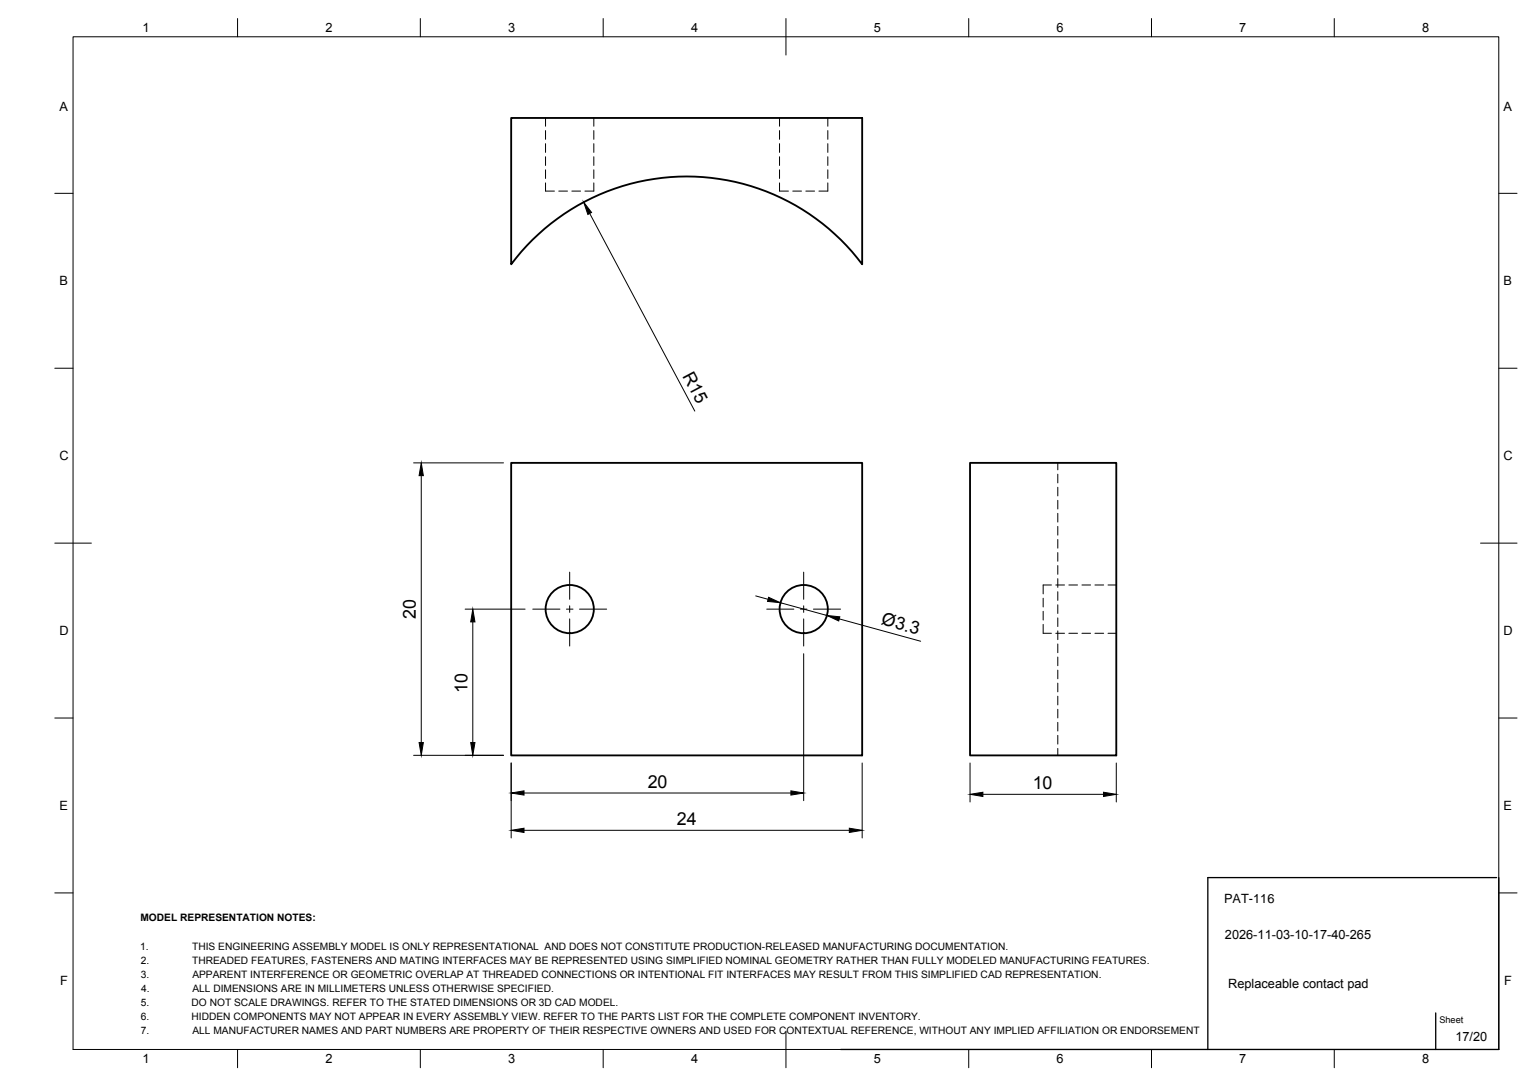
ISO-10303-21;
HEADER;
/* Generated by software containing ST-Developer
 * from STEP Tools, Inc. (www.steptools.com) 
 */

FILE_DESCRIPTION(
/* description */ ('V-block with clamp strap'),
/* implementation_level */ '2;1');

FILE_NAME(
/* name */ 'Replaceable contact pad.step',
/* time_stamp */ '2026-10-27T10:50:53-07:00',
/* author */ (''),
/* organization */ (''),
/* preprocessor_version */ 'ST-DEVELOPER v20.2',
/* originating_system */ 'Autodesk Translation Framework v15.17.0.0',
/* authorisation */ '');

FILE_SCHEMA (('AUTOMOTIVE_DESIGN { 1 0 10303 214 3 1 1 }'));
ENDSEC;

DATA;
#10=MECHANICAL_DESIGN_GEOMETRIC_PRESENTATION_REPRESENTATION('',(#280),#7344);
#238=SHAPE_REPRESENTATION_RELATIONSHIP('SRR','None',#7457,#259);
#259=ADVANCED_BREP_SHAPE_REPRESENTATION('',(#299),#7336);
#280=STYLED_ITEM('',(#7624),#299);
#299=MANIFOLD_SOLID_BREP('Body1',#4164);
#369=FACE_BOUND('',#1066,.T.);
#370=FACE_BOUND('',#1067,.T.);
#478=CIRCLE('',#4742,0.164999999999999);
#479=CIRCLE('',#4743,0.164999999999999);
#480=CIRCLE('',#4746,0.164999999999999);
#481=CIRCLE('',#4747,0.164999999999999);
#482=CIRCLE('',#4750,1.5);
#483=CIRCLE('',#4751,1.5);
#551=CYLINDRICAL_SURFACE('',#4741,0.164999999999999);
#552=CYLINDRICAL_SURFACE('',#4745,0.164999999999999);
#553=CYLINDRICAL_SURFACE('',#4749,1.5);
#752=FACE_OUTER_BOUND('',#1056,.T.);
#753=FACE_OUTER_BOUND('',#1057,.T.);
#754=FACE_OUTER_BOUND('',#1058,.T.);
#755=FACE_OUTER_BOUND('',#1059,.T.);
#756=FACE_OUTER_BOUND('',#1060,.T.);
#757=FACE_OUTER_BOUND('',#1061,.T.);
#758=FACE_OUTER_BOUND('',#1062,.T.);
#759=FACE_OUTER_BOUND('',#1063,.T.);
#760=FACE_OUTER_BOUND('',#1064,.T.);
#761=FACE_OUTER_BOUND('',#1065,.T.);
#1056=EDGE_LOOP('',(#3564,#3565,#3566,#3567));
#1057=EDGE_LOOP('',(#3568));
#1058=EDGE_LOOP('',(#3569,#3570,#3571,#3572));
#1059=EDGE_LOOP('',(#3573));
#1060=EDGE_LOOP('',(#3574,#3575,#3576,#3577));
#1061=EDGE_LOOP('',(#3578,#3579,#3580,#3581));
#1062=EDGE_LOOP('',(#3582,#3583,#3584,#3585));
#1063=EDGE_LOOP('',(#3586,#3587,#3588,#3589));
#1064=EDGE_LOOP('',(#3590,#3591,#3592,#3593));
#1065=EDGE_LOOP('',(#3594,#3595,#3596,#3597));
#1066=EDGE_LOOP('',(#3598));
#1067=EDGE_LOOP('',(#3599));
#1429=LINE('',#7053,#1794);
#1430=LINE('',#7060,#1795);
#1431=LINE('',#7066,#1796);
#1432=LINE('',#7070,#1797);
#1433=LINE('',#7074,#1798);
#1434=LINE('',#7076,#1799);
#1435=LINE('',#7077,#1800);
#1436=LINE('',#7080,#1801);
#1437=LINE('',#7081,#1802);
#1438=LINE('',#7084,#1803);
#1439=LINE('',#7085,#1804);
#1440=LINE('',#7087,#1805);
#1794=VECTOR('',#5837,0.164999999999999);
#1795=VECTOR('',#5846,0.164999999999999);
#1796=VECTOR('',#5853,1.);
#1797=VECTOR('',#5856,1.);
#1798=VECTOR('',#5861,1.);
#1799=VECTOR('',#5862,1.);
#1800=VECTOR('',#5863,1.);
#1801=VECTOR('',#5866,1.);
#1802=VECTOR('',#5867,1.);
#1803=VECTOR('',#5870,1.);
#1804=VECTOR('',#5871,1.);
#1805=VECTOR('',#5874,1.);
#2117=VERTEX_POINT('',#7050);
#2118=VERTEX_POINT('',#7052);
#2119=VERTEX_POINT('',#7057);
#2120=VERTEX_POINT('',#7059);
#2121=VERTEX_POINT('',#7064);
#2122=VERTEX_POINT('',#7065);
#2123=VERTEX_POINT('',#7067);
#2124=VERTEX_POINT('',#7069);
#2125=VERTEX_POINT('',#7073);
#2126=VERTEX_POINT('',#7075);
#2127=VERTEX_POINT('',#7079);
#2128=VERTEX_POINT('',#7083);
#2608=EDGE_CURVE('',#2117,#2117,#478,.T.);
#2609=EDGE_CURVE('',#2117,#2118,#1429,.T.);
#2610=EDGE_CURVE('',#2118,#2118,#479,.T.);
#2611=EDGE_CURVE('',#2119,#2119,#480,.T.);
#2612=EDGE_CURVE('',#2119,#2120,#1430,.T.);
#2613=EDGE_CURVE('',#2120,#2120,#481,.T.);
#2614=EDGE_CURVE('',#2121,#2122,#1431,.T.);
#2615=EDGE_CURVE('',#2123,#2121,#482,.T.);
#2616=EDGE_CURVE('',#2124,#2123,#1432,.T.);
#2617=EDGE_CURVE('',#2122,#2124,#483,.T.);
#2618=EDGE_CURVE('',#2121,#2125,#1433,.T.);
#2619=EDGE_CURVE('',#2126,#2125,#1434,.T.);
#2620=EDGE_CURVE('',#2123,#2126,#1435,.T.);
#2621=EDGE_CURVE('',#2122,#2127,#1436,.T.);
#2622=EDGE_CURVE('',#2125,#2127,#1437,.T.);
#2623=EDGE_CURVE('',#2128,#2126,#1438,.T.);
#2624=EDGE_CURVE('',#2124,#2128,#1439,.T.);
#2625=EDGE_CURVE('',#2127,#2128,#1440,.T.);
#3564=ORIENTED_EDGE('',*,*,#2608,.F.);
#3565=ORIENTED_EDGE('',*,*,#2609,.T.);
#3566=ORIENTED_EDGE('',*,*,#2610,.F.);
#3567=ORIENTED_EDGE('',*,*,#2609,.F.);
#3568=ORIENTED_EDGE('',*,*,#2608,.T.);
#3569=ORIENTED_EDGE('',*,*,#2611,.F.);
#3570=ORIENTED_EDGE('',*,*,#2612,.T.);
#3571=ORIENTED_EDGE('',*,*,#2613,.F.);
#3572=ORIENTED_EDGE('',*,*,#2612,.F.);
#3573=ORIENTED_EDGE('',*,*,#2611,.T.);
#3574=ORIENTED_EDGE('',*,*,#2614,.F.);
#3575=ORIENTED_EDGE('',*,*,#2615,.F.);
#3576=ORIENTED_EDGE('',*,*,#2616,.F.);
#3577=ORIENTED_EDGE('',*,*,#2617,.F.);
#3578=ORIENTED_EDGE('',*,*,#2615,.T.);
#3579=ORIENTED_EDGE('',*,*,#2618,.T.);
#3580=ORIENTED_EDGE('',*,*,#2619,.F.);
#3581=ORIENTED_EDGE('',*,*,#2620,.F.);
#3582=ORIENTED_EDGE('',*,*,#2614,.T.);
#3583=ORIENTED_EDGE('',*,*,#2621,.T.);
#3584=ORIENTED_EDGE('',*,*,#2622,.F.);
#3585=ORIENTED_EDGE('',*,*,#2618,.F.);
#3586=ORIENTED_EDGE('',*,*,#2616,.T.);
#3587=ORIENTED_EDGE('',*,*,#2620,.T.);
#3588=ORIENTED_EDGE('',*,*,#2623,.F.);
#3589=ORIENTED_EDGE('',*,*,#2624,.F.);
#3590=ORIENTED_EDGE('',*,*,#2617,.T.);
#3591=ORIENTED_EDGE('',*,*,#2624,.T.);
#3592=ORIENTED_EDGE('',*,*,#2625,.F.);
#3593=ORIENTED_EDGE('',*,*,#2621,.F.);
#3594=ORIENTED_EDGE('',*,*,#2625,.T.);
#3595=ORIENTED_EDGE('',*,*,#2623,.T.);
#3596=ORIENTED_EDGE('',*,*,#2619,.T.);
#3597=ORIENTED_EDGE('',*,*,#2622,.T.);
#3598=ORIENTED_EDGE('',*,*,#2610,.T.);
#3599=ORIENTED_EDGE('',*,*,#2613,.T.);
#3874=PLANE('',#4744);
#3875=PLANE('',#4748);
#3876=PLANE('',#4752);
#3877=PLANE('',#4753);
#3878=PLANE('',#4754);
#3879=PLANE('',#4755);
#3880=PLANE('',#4756);
#4098=ADVANCED_FACE('',(#752),#551,.F.);
#4099=ADVANCED_FACE('',(#753),#3874,.T.);
#4100=ADVANCED_FACE('',(#754),#552,.F.);
#4101=ADVANCED_FACE('',(#755),#3875,.T.);
#4102=ADVANCED_FACE('',(#756),#553,.F.);
#4103=ADVANCED_FACE('',(#757),#3876,.T.);
#4104=ADVANCED_FACE('',(#758),#3877,.T.);
#4105=ADVANCED_FACE('',(#759),#3878,.T.);
#4106=ADVANCED_FACE('',(#760),#3879,.T.);
#4107=ADVANCED_FACE('',(#761,#369,#370),#3880,.T.);
#4164=CLOSED_SHELL('',(#4098,#4099,#4100,#4101,#4102,#4103,#4104,#4105,
#4106,#4107));
#4740=AXIS2_PLACEMENT_3D('',#7048,#5831,#5832);
#4741=AXIS2_PLACEMENT_3D('',#7049,#5833,#5834);
#4742=AXIS2_PLACEMENT_3D('',#7051,#5835,#5836);
#4743=AXIS2_PLACEMENT_3D('',#7054,#5838,#5839);
#4744=AXIS2_PLACEMENT_3D('',#7055,#5840,#5841);
#4745=AXIS2_PLACEMENT_3D('',#7056,#5842,#5843);
#4746=AXIS2_PLACEMENT_3D('',#7058,#5844,#5845);
#4747=AXIS2_PLACEMENT_3D('',#7061,#5847,#5848);
#4748=AXIS2_PLACEMENT_3D('',#7062,#5849,#5850);
#4749=AXIS2_PLACEMENT_3D('',#7063,#5851,#5852);
#4750=AXIS2_PLACEMENT_3D('',#7068,#5854,#5855);
#4751=AXIS2_PLACEMENT_3D('',#7071,#5857,#5858);
#4752=AXIS2_PLACEMENT_3D('',#7072,#5859,#5860);
#4753=AXIS2_PLACEMENT_3D('',#7078,#5864,#5865);
#4754=AXIS2_PLACEMENT_3D('',#7082,#5868,#5869);
#4755=AXIS2_PLACEMENT_3D('',#7086,#5872,#5873);
#4756=AXIS2_PLACEMENT_3D('',#7088,#5875,#5876);
#5831=DIRECTION('axis',(0.,0.,1.));
#5832=DIRECTION('refdir',(1.,0.,0.));
#5833=DIRECTION('center_axis',(0.,0.,1.));
#5834=DIRECTION('ref_axis',(1.,0.,0.));
#5835=DIRECTION('center_axis',(0.,0.,1.));
#5836=DIRECTION('ref_axis',(1.,0.,0.));
#5837=DIRECTION('',(0.,0.,1.));
#5838=DIRECTION('center_axis',(0.,0.,-1.));
#5839=DIRECTION('ref_axis',(1.,0.,0.));
#5840=DIRECTION('center_axis',(0.,0.,1.));
#5841=DIRECTION('ref_axis',(1.,0.,0.));
#5842=DIRECTION('center_axis',(0.,0.,1.));
#5843=DIRECTION('ref_axis',(1.,0.,0.));
#5844=DIRECTION('center_axis',(0.,0.,1.));
#5845=DIRECTION('ref_axis',(1.,0.,0.));
#5846=DIRECTION('',(0.,0.,1.));
#5847=DIRECTION('center_axis',(0.,0.,-1.));
#5848=DIRECTION('ref_axis',(1.,0.,0.));
#5849=DIRECTION('center_axis',(0.,0.,1.));
#5850=DIRECTION('ref_axis',(1.,0.,0.));
#5851=DIRECTION('center_axis',(1.,0.,0.));
#5852=DIRECTION('ref_axis',(0.,1.22464679914735E-16,1.));
#5853=DIRECTION('',(-1.,0.,0.));
#5854=DIRECTION('center_axis',(-1.,0.,0.));
#5855=DIRECTION('ref_axis',(0.,0.,-1.));
#5856=DIRECTION('',(1.,0.,0.));
#5857=DIRECTION('center_axis',(1.,0.,0.));
#5858=DIRECTION('ref_axis',(0.,0.,-1.));
#5859=DIRECTION('center_axis',(1.,0.,0.));
#5860=DIRECTION('ref_axis',(0.,1.,0.));
#5861=DIRECTION('',(0.,0.,1.));
#5862=DIRECTION('',(0.,1.,0.));
#5863=DIRECTION('',(0.,0.,1.));
#5864=DIRECTION('center_axis',(0.,1.,0.));
#5865=DIRECTION('ref_axis',(-1.,0.,0.));
#5866=DIRECTION('',(0.,0.,1.));
#5867=DIRECTION('',(-1.,0.,0.));
#5868=DIRECTION('center_axis',(0.,-1.,0.));
#5869=DIRECTION('ref_axis',(1.,0.,0.));
#5870=DIRECTION('',(1.,0.,0.));
#5871=DIRECTION('',(0.,0.,1.));
#5872=DIRECTION('center_axis',(-1.,0.,0.));
#5873=DIRECTION('ref_axis',(0.,-1.,0.));
#5874=DIRECTION('',(0.,-1.,0.));
#5875=DIRECTION('center_axis',(0.,0.,1.));
#5876=DIRECTION('ref_axis',(1.,0.,0.));
#7048=CARTESIAN_POINT('',(0.,0.,0.));
#7049=CARTESIAN_POINT('Origin',(10.,-0.8,6.02132034));
#7050=CARTESIAN_POINT('',(9.835,-0.8,6.02132034));
#7051=CARTESIAN_POINT('Origin',(10.,-0.8,6.02132034));
#7052=CARTESIAN_POINT('',(9.835,-0.8,6.52132034));
#7053=CARTESIAN_POINT('',(9.835,-0.8,6.02132034));
#7054=CARTESIAN_POINT('Origin',(10.,-0.8,6.52132034));
#7055=CARTESIAN_POINT('Origin',(10.,-0.8,6.02132034));
#7056=CARTESIAN_POINT('Origin',(10.,0.8,6.02132034));
#7057=CARTESIAN_POINT('',(9.835,0.8,6.02132034));
#7058=CARTESIAN_POINT('Origin',(10.,0.8,6.02132034));
#7059=CARTESIAN_POINT('',(9.835,0.8,6.52132034));
#7060=CARTESIAN_POINT('',(9.835,0.8,6.02132034));
#7061=CARTESIAN_POINT('Origin',(10.,0.8,6.52132034));
#7062=CARTESIAN_POINT('Origin',(10.,0.8,6.02132034));
#7063=CARTESIAN_POINT('Origin',(8.9,0.,4.62132034355964));
#7064=CARTESIAN_POINT('',(11.,1.2,5.52132034));
#7065=CARTESIAN_POINT('',(9.,1.2,5.52132034));
#7066=CARTESIAN_POINT('',(11.,1.2,5.52132034));
#7067=CARTESIAN_POINT('',(11.,-1.2,5.52132034));
#7068=CARTESIAN_POINT('Origin',(11.,0.,4.62132034355964));
#7069=CARTESIAN_POINT('',(9.,-1.2,5.52132034));
#7070=CARTESIAN_POINT('',(9.,-1.2,5.52132034));
#7071=CARTESIAN_POINT('Origin',(9.,0.,4.62132034355964));
#7072=CARTESIAN_POINT('Origin',(11.,-1.2,5.52132034));
#7073=CARTESIAN_POINT('',(11.,1.2,6.52132034));
#7074=CARTESIAN_POINT('',(11.,1.2,5.52132034));
#7075=CARTESIAN_POINT('',(11.,-1.2,6.52132034));
#7076=CARTESIAN_POINT('',(11.,-1.2,6.52132034));
#7077=CARTESIAN_POINT('',(11.,-1.2,5.52132034));
#7078=CARTESIAN_POINT('Origin',(11.,1.2,5.52132034));
#7079=CARTESIAN_POINT('',(9.,1.2,6.52132034));
#7080=CARTESIAN_POINT('',(9.,1.2,5.52132034));
#7081=CARTESIAN_POINT('',(11.,1.2,6.52132034));
#7082=CARTESIAN_POINT('Origin',(9.,-1.2,5.52132034));
#7083=CARTESIAN_POINT('',(9.,-1.2,6.52132034));
#7084=CARTESIAN_POINT('',(9.,-1.2,6.52132034));
#7085=CARTESIAN_POINT('',(9.,-1.2,5.52132034));
#7086=CARTESIAN_POINT('Origin',(9.,1.2,5.52132034));
#7087=CARTESIAN_POINT('',(9.,1.2,6.52132034));
#7088=CARTESIAN_POINT('Origin',(10.,0.,6.52132034));
#7310=UNCERTAINTY_MEASURE_WITH_UNIT(LENGTH_MEASURE(0.001),#7345,
'DISTANCE_ACCURACY_VALUE',
'Maximum model space distance between geometric entities at asserted c
onnectivities');
#7318=UNCERTAINTY_MEASURE_WITH_UNIT(LENGTH_MEASURE(0.001),#7345,
'DISTANCE_ACCURACY_VALUE',
'Maximum model space distance between geometric entities at asserted c
onnectivities');
#7336=(
GEOMETRIC_REPRESENTATION_CONTEXT(3)
GLOBAL_UNCERTAINTY_ASSIGNED_CONTEXT((#7310))
GLOBAL_UNIT_ASSIGNED_CONTEXT((#7345,#7347,#7348))
REPRESENTATION_CONTEXT('','3D')
);
#7344=(
GEOMETRIC_REPRESENTATION_CONTEXT(3)
GLOBAL_UNCERTAINTY_ASSIGNED_CONTEXT((#7318))
GLOBAL_UNIT_ASSIGNED_CONTEXT((#7345,#7347,#7348))
REPRESENTATION_CONTEXT('','3D')
);
#7345=(
LENGTH_UNIT()
NAMED_UNIT(*)
SI_UNIT(.CENTI.,.METRE.)
);
#7347=(
NAMED_UNIT(*)
PLANE_ANGLE_UNIT()
SI_UNIT($,.RADIAN.)
);
#7348=(
NAMED_UNIT(*)
SI_UNIT($,.STERADIAN.)
SOLID_ANGLE_UNIT()
);
#7366=SHAPE_DEFINITION_REPRESENTATION(#7414,#7457);
#7414=PRODUCT_DEFINITION_SHAPE('',$,#7483);
#7457=SHAPE_REPRESENTATION('',(#4740),#7336);
#7465=PRODUCT_DEFINITION_CONTEXT('part definition',#7542,'design');
#7483=PRODUCT_DEFINITION('Replaceable contact pad',
'Replaceable contact pad',#7508,#7465);
#7508=PRODUCT_DEFINITION_FORMATION('',$,#7561);
#7542=APPLICATION_CONTEXT(
'Core Data for Automotive Mechanical Design Process');
#7543=PRODUCT_CONTEXT('part definition',#7542,'mechanical');
#7561=PRODUCT('Replaceable contact pad','Replaceable contact pad',
'Replaceable contact pad',(#7543));
#7618=COLOUR_RGB('Sky Blue',0.24,0.69,0.87);
#7619=FILL_AREA_STYLE_COLOUR('',#7618);
#7620=FILL_AREA_STYLE('',(#7619));
#7621=SURFACE_STYLE_FILL_AREA(#7620);
#7622=SURFACE_SIDE_STYLE('',(#7621));
#7623=SURFACE_STYLE_USAGE(.BOTH.,#7622);
#7624=PRESENTATION_STYLE_ASSIGNMENT((#7623));
ENDSEC;
END-ISO-10303-21;
